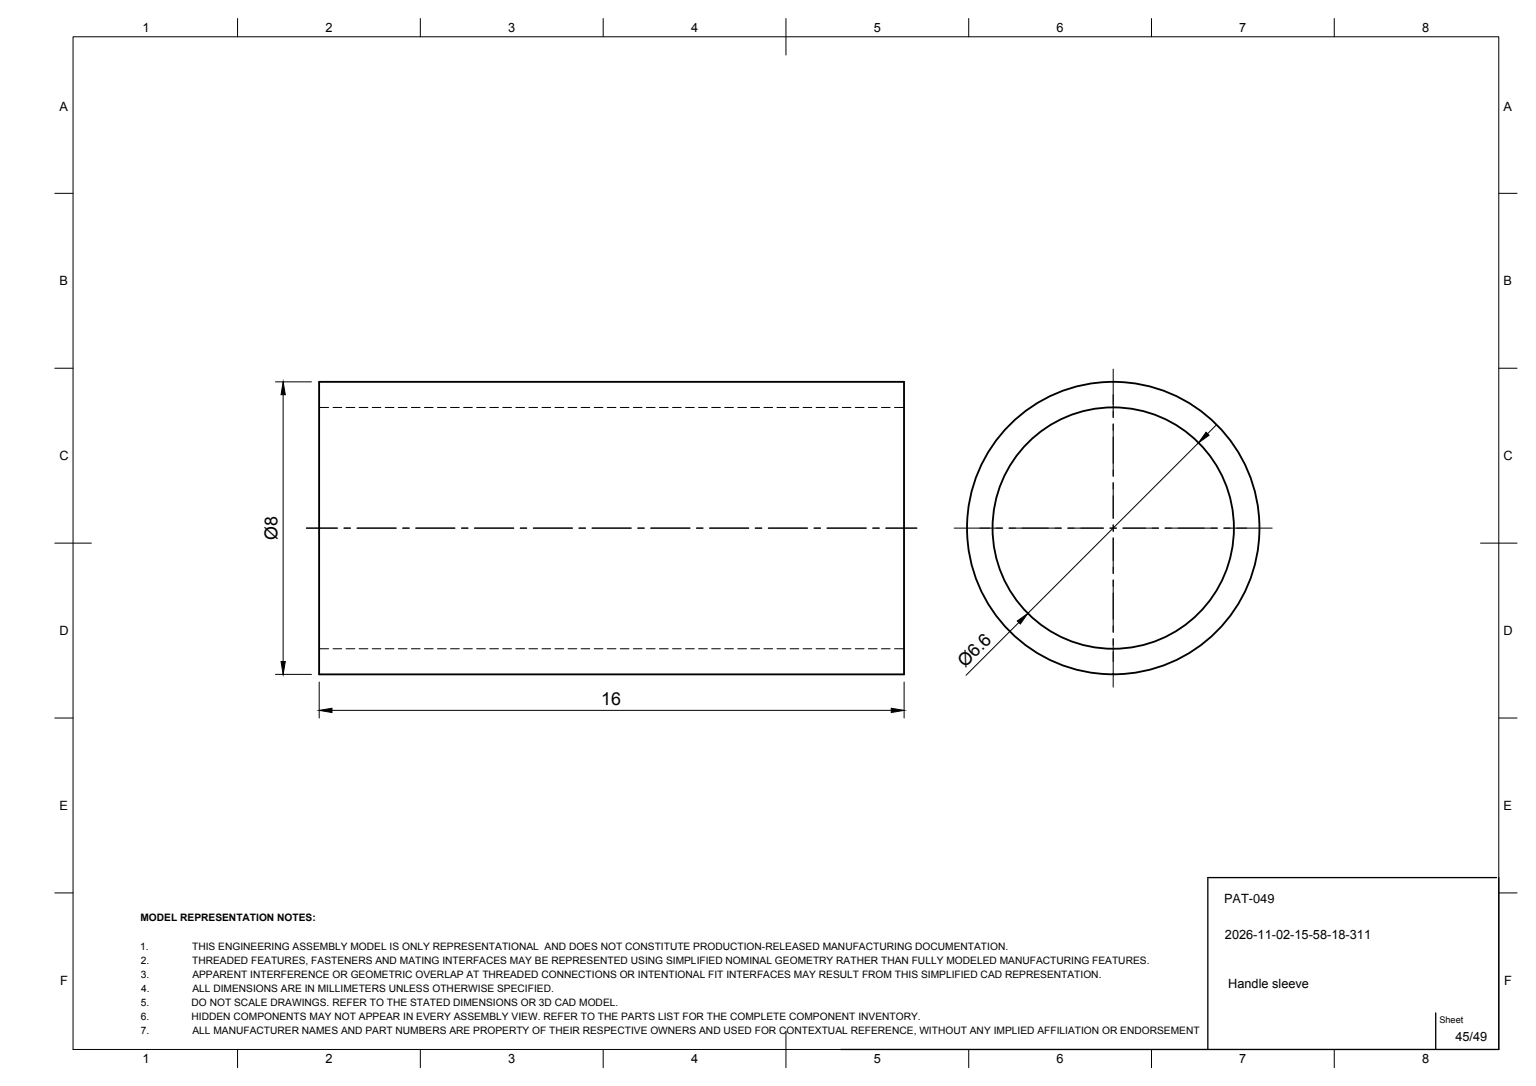
ISO-10303-21;
HEADER;
/* Generated by software containing ST-Developer
 * from STEP Tools, Inc. (www.steptools.com) 
 */

FILE_DESCRIPTION(
/* description */ ('Hand drill press frame (manual)'),
/* implementation_level */ '2;1');

FILE_NAME(
/* name */ 'Handle sleeve.step',
/* time_stamp */ '2026-10-28T03:25:28-07:00',
/* author */ (''),
/* organization */ (''),
/* preprocessor_version */ 'ST-DEVELOPER v20.2',
/* originating_system */ 'Autodesk Translation Framework v15.17.0.0',
/* authorisation */ '');

FILE_SCHEMA (('AUTOMOTIVE_DESIGN { 1 0 10303 214 3 1 1 }'));
ENDSEC;

DATA;
#10=MECHANICAL_DESIGN_GEOMETRIC_PRESENTATION_REPRESENTATION('',(#663),#33299);
#566=SHAPE_REPRESENTATION_RELATIONSHIP('SRR','None',#33528,#611);
#611=ADVANCED_BREP_SHAPE_REPRESENTATION('',(#714),#33290);
#663=STYLED_ITEM('',(#33828),#714);
#714=MANIFOLD_SOLID_BREP('Body1',#12682);
#872=FACE_BOUND('',#2730,.T.);
#873=FACE_BOUND('',#2732,.T.);
#1281=PLANE('',#14114);
#1282=PLANE('',#14115);
#1886=FACE_OUTER_BOUND('',#2727,.T.);
#1887=FACE_OUTER_BOUND('',#2728,.T.);
#1888=FACE_OUTER_BOUND('',#2729,.T.);
#1889=FACE_OUTER_BOUND('',#2731,.T.);
#2727=EDGE_LOOP('',(#11087,#11088,#11089,#11090));
#2728=EDGE_LOOP('',(#11091,#11092,#11093,#11094));
#2729=EDGE_LOOP('',(#11095));
#2730=EDGE_LOOP('',(#11096));
#2731=EDGE_LOOP('',(#11097));
#2732=EDGE_LOOP('',(#11098));
#3860=LINE('',#21322,#5025);
#3861=LINE('',#21328,#5026);
#5025=VECTOR('',#17187,0.33);
#5026=VECTOR('',#17194,0.4);
#5533=CIRCLE('',#14109,0.33);
#5534=CIRCLE('',#14110,0.33);
#5535=CIRCLE('',#14112,0.4);
#5536=CIRCLE('',#14113,0.4);
#6509=VERTEX_POINT('',#21319);
#6510=VERTEX_POINT('',#21321);
#6511=VERTEX_POINT('',#21325);
#6512=VERTEX_POINT('',#21327);
#8072=EDGE_CURVE('',#6509,#6509,#5533,.T.);
#8073=EDGE_CURVE('',#6509,#6510,#3860,.T.);
#8074=EDGE_CURVE('',#6510,#6510,#5534,.T.);
#8075=EDGE_CURVE('',#6511,#6511,#5535,.T.);
#8076=EDGE_CURVE('',#6511,#6512,#3861,.T.);
#8077=EDGE_CURVE('',#6512,#6512,#5536,.T.);
#11087=ORIENTED_EDGE('',*,*,#8072,.F.);
#11088=ORIENTED_EDGE('',*,*,#8073,.T.);
#11089=ORIENTED_EDGE('',*,*,#8074,.T.);
#11090=ORIENTED_EDGE('',*,*,#8073,.F.);
#11091=ORIENTED_EDGE('',*,*,#8075,.F.);
#11092=ORIENTED_EDGE('',*,*,#8076,.T.);
#11093=ORIENTED_EDGE('',*,*,#8077,.T.);
#11094=ORIENTED_EDGE('',*,*,#8076,.F.);
#11095=ORIENTED_EDGE('',*,*,#8075,.T.);
#11096=ORIENTED_EDGE('',*,*,#8072,.T.);
#11097=ORIENTED_EDGE('',*,*,#8077,.F.);
#11098=ORIENTED_EDGE('',*,*,#8074,.F.);
#11912=CYLINDRICAL_SURFACE('',#14108,0.33);
#11913=CYLINDRICAL_SURFACE('',#14111,0.4);
#12495=ADVANCED_FACE('',(#1886),#11912,.F.);
#12496=ADVANCED_FACE('',(#1887),#11913,.T.);
#12497=ADVANCED_FACE('',(#1888,#872),#1281,.T.);
#12498=ADVANCED_FACE('',(#1889,#873),#1282,.F.);
#12682=CLOSED_SHELL('',(#12495,#12496,#12497,#12498));
#14107=AXIS2_PLACEMENT_3D('',#21317,#17181,#17182);
#14108=AXIS2_PLACEMENT_3D('',#21318,#17183,#17184);
#14109=AXIS2_PLACEMENT_3D('',#21320,#17185,#17186);
#14110=AXIS2_PLACEMENT_3D('',#21323,#17188,#17189);
#14111=AXIS2_PLACEMENT_3D('',#21324,#17190,#17191);
#14112=AXIS2_PLACEMENT_3D('',#21326,#17192,#17193);
#14113=AXIS2_PLACEMENT_3D('',#21329,#17195,#17196);
#14114=AXIS2_PLACEMENT_3D('',#21330,#17197,#17198);
#14115=AXIS2_PLACEMENT_3D('',#21331,#17199,#17200);
#17181=DIRECTION('axis',(0.,0.,1.));
#17182=DIRECTION('refdir',(1.,0.,0.));
#17183=DIRECTION('center_axis',(0.,1.,0.));
#17184=DIRECTION('ref_axis',(1.,0.,0.));
#17185=DIRECTION('center_axis',(0.,-1.,0.));
#17186=DIRECTION('ref_axis',(1.,0.,0.));
#17187=DIRECTION('',(0.,-1.,0.));
#17188=DIRECTION('center_axis',(0.,-1.,0.));
#17189=DIRECTION('ref_axis',(1.,0.,0.));
#17190=DIRECTION('center_axis',(0.,1.,0.));
#17191=DIRECTION('ref_axis',(1.,0.,0.));
#17192=DIRECTION('center_axis',(0.,1.,0.));
#17193=DIRECTION('ref_axis',(1.,0.,0.));
#17194=DIRECTION('',(0.,-1.,0.));
#17195=DIRECTION('center_axis',(0.,1.,0.));
#17196=DIRECTION('ref_axis',(1.,0.,0.));
#17197=DIRECTION('center_axis',(0.,1.,0.));
#17198=DIRECTION('ref_axis',(1.,0.,0.));
#17199=DIRECTION('center_axis',(0.,1.,0.));
#17200=DIRECTION('ref_axis',(1.,0.,0.));
#21317=CARTESIAN_POINT('',(0.,0.,0.));
#21318=CARTESIAN_POINT('Origin',(-3.25,6.8,29.));
#21319=CARTESIAN_POINT('',(-3.58,8.4,29.));
#21320=CARTESIAN_POINT('Origin',(-3.25,8.4,29.));
#21321=CARTESIAN_POINT('',(-3.58,6.8,29.));
#21322=CARTESIAN_POINT('',(-3.58,6.8,29.));
#21323=CARTESIAN_POINT('Origin',(-3.25,6.8,29.));
#21324=CARTESIAN_POINT('Origin',(-3.25,6.8,29.));
#21325=CARTESIAN_POINT('',(-3.65,8.4,29.));
#21326=CARTESIAN_POINT('Origin',(-3.25,8.4,29.));
#21327=CARTESIAN_POINT('',(-3.65,6.8,29.));
#21328=CARTESIAN_POINT('',(-3.65,6.8,29.));
#21329=CARTESIAN_POINT('Origin',(-3.25,6.8,29.));
#21330=CARTESIAN_POINT('Origin',(-3.25,8.4,29.));
#21331=CARTESIAN_POINT('Origin',(-3.25,6.8,29.));
#33238=UNCERTAINTY_MEASURE_WITH_UNIT(LENGTH_MEASURE(0.001),#33300,
'DISTANCE_ACCURACY_VALUE',
'Maximum model space distance between geometric entities at asserted c
onnectivities');
#33247=UNCERTAINTY_MEASURE_WITH_UNIT(LENGTH_MEASURE(0.001),#33300,
'DISTANCE_ACCURACY_VALUE',
'Maximum model space distance between geometric entities at asserted c
onnectivities');
#33290=(
GEOMETRIC_REPRESENTATION_CONTEXT(3)
GLOBAL_UNCERTAINTY_ASSIGNED_CONTEXT((#33238))
GLOBAL_UNIT_ASSIGNED_CONTEXT((#33300,#33302,#33303))
REPRESENTATION_CONTEXT('','3D')
);
#33299=(
GEOMETRIC_REPRESENTATION_CONTEXT(3)
GLOBAL_UNCERTAINTY_ASSIGNED_CONTEXT((#33247))
GLOBAL_UNIT_ASSIGNED_CONTEXT((#33300,#33302,#33303))
REPRESENTATION_CONTEXT('','3D')
);
#33300=(
LENGTH_UNIT()
NAMED_UNIT(*)
SI_UNIT(.CENTI.,.METRE.)
);
#33302=(
NAMED_UNIT(*)
PLANE_ANGLE_UNIT()
SI_UNIT($,.RADIAN.)
);
#33303=(
NAMED_UNIT(*)
SI_UNIT($,.STERADIAN.)
SOLID_ANGLE_UNIT()
);
#33346=SHAPE_DEFINITION_REPRESENTATION(#33408,#33528);
#33408=PRODUCT_DEFINITION_SHAPE('',$,#33580);
#33528=SHAPE_REPRESENTATION('',(#14107),#33290);
#33537=PRODUCT_DEFINITION_CONTEXT('part definition',#33692,'design');
#33580=PRODUCT_DEFINITION('Handle sleeve','Handle sleeve',#33631,#33537);
#33631=PRODUCT_DEFINITION_FORMATION('',$,#33736);
#33692=APPLICATION_CONTEXT(
'Core Data for Automotive Mechanical Design Process');
#33693=PRODUCT_CONTEXT('part definition',#33692,'mechanical');
#33736=PRODUCT('Handle sleeve','Handle sleeve','Handle sleeve',(#33693));
#33822=COLOUR_RGB('Off White',0.89,0.88,0.83);
#33823=FILL_AREA_STYLE_COLOUR('',#33822);
#33824=FILL_AREA_STYLE('',(#33823));
#33825=SURFACE_STYLE_FILL_AREA(#33824);
#33826=SURFACE_SIDE_STYLE('',(#33825));
#33827=SURFACE_STYLE_USAGE(.BOTH.,#33826);
#33828=PRESENTATION_STYLE_ASSIGNMENT((#33827));
ENDSEC;
END-ISO-10303-21;
